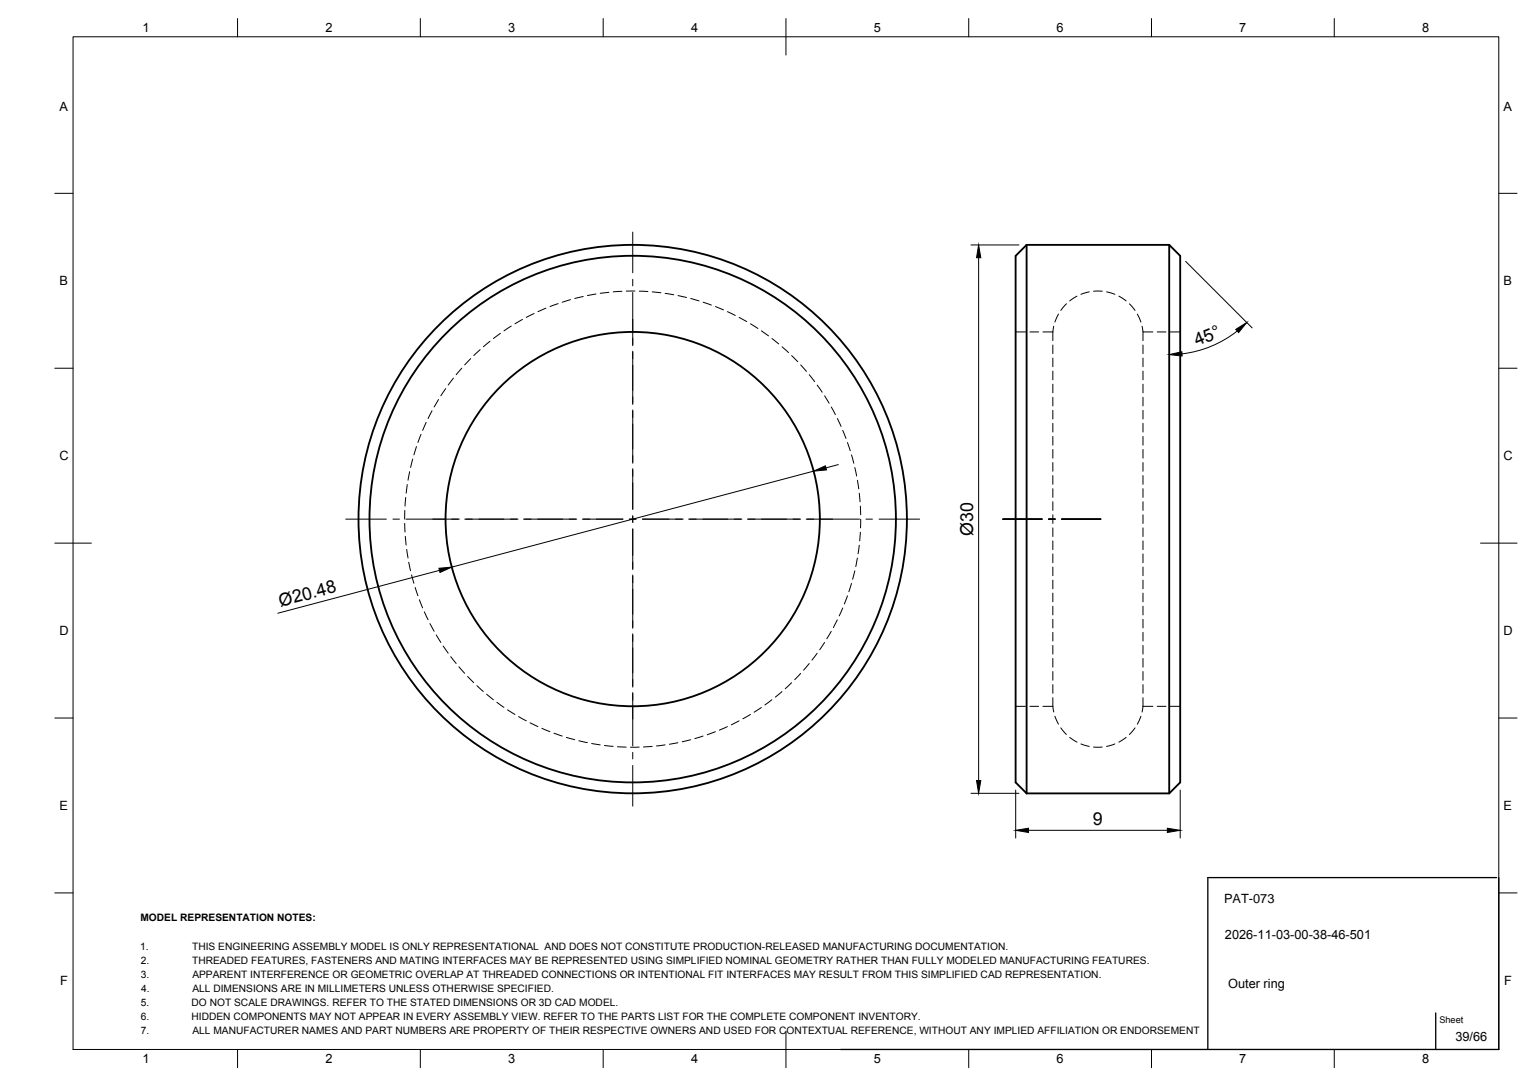
ISO-10303-21;
HEADER;
/* Generated by software containing ST-Developer
 * from STEP Tools, Inc. (www.steptools.com) 
 */

FILE_DESCRIPTION(
/* description */ ('Manual piston pump'),
/* implementation_level */ '2;1');

FILE_NAME(
/* name */ 'Outer ring.step',
/* time_stamp */ '2026-11-02T16:54:23-08:00',
/* author */ (''),
/* organization */ (''),
/* preprocessor_version */ 'ST-DEVELOPER v20.2',
/* originating_system */ 'Autodesk Translation Framework v15.17.0.0',
/* authorisation */ '');

FILE_SCHEMA (('AUTOMOTIVE_DESIGN { 1 0 10303 214 3 1 1 }'));
ENDSEC;

DATA;
#10=MECHANICAL_DESIGN_GEOMETRIC_PRESENTATION_REPRESENTATION('',(#712),#19043);
#539=CONICAL_SURFACE('',#10737,1.47,0.785398163397449);
#540=CONICAL_SURFACE('',#10741,1.47,0.785398163397449);
#560=TOROIDAL_SURFACE('',#10726,1.,0.247676);
#586=SHAPE_REPRESENTATION_RELATIONSHIP('SRR','None',#19333,#649);
#649=ADVANCED_BREP_SHAPE_REPRESENTATION('',(#782),#19000);
#712=STYLED_ITEM('',(#19664),#782);
#782=MANIFOLD_SOLID_BREP('Body1',#9498);
#948=FACE_BOUND('',#2237,.T.);
#949=FACE_BOUND('',#2242,.T.);
#1186=CYLINDRICAL_SURFACE('',#10732,1.023815);
#1187=CYLINDRICAL_SURFACE('',#10739,1.5);
#1188=CYLINDRICAL_SURFACE('',#10744,1.023815);
#1538=FACE_OUTER_BOUND('',#2234,.T.);
#1539=FACE_OUTER_BOUND('',#2235,.T.);
#1540=FACE_OUTER_BOUND('',#2236,.T.);
#1541=FACE_OUTER_BOUND('',#2238,.T.);
#1542=FACE_OUTER_BOUND('',#2239,.T.);
#1543=FACE_OUTER_BOUND('',#2240,.T.);
#1544=FACE_OUTER_BOUND('',#2241,.T.);
#1545=FACE_OUTER_BOUND('',#2243,.T.);
#2234=EDGE_LOOP('',(#7281,#7282,#7283,#7284,#7285,#7286));
#2235=EDGE_LOOP('',(#7287,#7288,#7289,#7290,#7291));
#2236=EDGE_LOOP('',(#7292));
#2237=EDGE_LOOP('',(#7293));
#2238=EDGE_LOOP('',(#7294,#7295,#7296,#7297));
#2239=EDGE_LOOP('',(#7298,#7299,#7300,#7301));
#2240=EDGE_LOOP('',(#7302,#7303,#7304,#7305));
#2241=EDGE_LOOP('',(#7306));
#2242=EDGE_LOOP('',(#7307));
#2243=EDGE_LOOP('',(#7308,#7309,#7310,#7311,#7312));
#2872=CIRCLE('',#10727,1.023815);
#2873=CIRCLE('',#10728,1.023815);
#2874=CIRCLE('',#10729,0.247676);
#2875=CIRCLE('',#10730,1.023815);
#2876=CIRCLE('',#10731,1.023815);
#2877=CIRCLE('',#10733,1.023815);
#2878=CIRCLE('',#10735,1.44);
#2879=CIRCLE('',#10736,1.023815);
#2880=CIRCLE('',#10738,1.5);
#2881=CIRCLE('',#10740,1.5);
#2882=CIRCLE('',#10742,1.44);
#3427=LINE('',#15800,#4031);
#3428=LINE('',#15809,#4032);
#3429=LINE('',#15813,#4033);
#3430=LINE('',#15817,#4034);
#3431=LINE('',#15820,#4035);
#4031=VECTOR('',#12757,1.023815);
#4032=VECTOR('',#12768,1.47);
#4033=VECTOR('',#12773,1.5);
#4034=VECTOR('',#12778,1.47);
#4035=VECTOR('',#12783,1.023815);
#4686=VERTEX_POINT('',#15788);
#4687=VERTEX_POINT('',#15789);
#4688=VERTEX_POINT('',#15792);
#4689=VERTEX_POINT('',#15794);
#4690=VERTEX_POINT('',#15798);
#4691=VERTEX_POINT('',#15802);
#4692=VERTEX_POINT('',#15804);
#4693=VERTEX_POINT('',#15807);
#4694=VERTEX_POINT('',#15811);
#4695=VERTEX_POINT('',#15815);
#5627=EDGE_CURVE('',#4686,#4687,#2872,.T.);
#5628=EDGE_CURVE('',#4687,#4686,#2873,.T.);
#5629=EDGE_CURVE('',#4687,#4688,#2874,.T.);
#5630=EDGE_CURVE('',#4689,#4688,#2875,.T.);
#5631=EDGE_CURVE('',#4688,#4689,#2876,.T.);
#5632=EDGE_CURVE('',#4690,#4690,#2877,.T.);
#5633=EDGE_CURVE('',#4690,#4689,#3427,.T.);
#5634=EDGE_CURVE('',#4691,#4691,#2878,.T.);
#5635=EDGE_CURVE('',#4692,#4692,#2879,.T.);
#5636=EDGE_CURVE('',#4693,#4693,#2880,.T.);
#5637=EDGE_CURVE('',#4693,#4691,#3428,.T.);
#5638=EDGE_CURVE('',#4694,#4694,#2881,.T.);
#5639=EDGE_CURVE('',#4694,#4693,#3429,.T.);
#5640=EDGE_CURVE('',#4695,#4695,#2882,.T.);
#5641=EDGE_CURVE('',#4695,#4694,#3430,.T.);
#5642=EDGE_CURVE('',#4686,#4692,#3431,.T.);
#7281=ORIENTED_EDGE('',*,*,#5627,.F.);
#7282=ORIENTED_EDGE('',*,*,#5628,.F.);
#7283=ORIENTED_EDGE('',*,*,#5629,.T.);
#7284=ORIENTED_EDGE('',*,*,#5630,.F.);
#7285=ORIENTED_EDGE('',*,*,#5631,.F.);
#7286=ORIENTED_EDGE('',*,*,#5629,.F.);
#7287=ORIENTED_EDGE('',*,*,#5632,.T.);
#7288=ORIENTED_EDGE('',*,*,#5633,.T.);
#7289=ORIENTED_EDGE('',*,*,#5630,.T.);
#7290=ORIENTED_EDGE('',*,*,#5631,.T.);
#7291=ORIENTED_EDGE('',*,*,#5633,.F.);
#7292=ORIENTED_EDGE('',*,*,#5634,.F.);
#7293=ORIENTED_EDGE('',*,*,#5635,.T.);
#7294=ORIENTED_EDGE('',*,*,#5636,.F.);
#7295=ORIENTED_EDGE('',*,*,#5637,.T.);
#7296=ORIENTED_EDGE('',*,*,#5634,.T.);
#7297=ORIENTED_EDGE('',*,*,#5637,.F.);
#7298=ORIENTED_EDGE('',*,*,#5638,.F.);
#7299=ORIENTED_EDGE('',*,*,#5639,.T.);
#7300=ORIENTED_EDGE('',*,*,#5636,.T.);
#7301=ORIENTED_EDGE('',*,*,#5639,.F.);
#7302=ORIENTED_EDGE('',*,*,#5640,.F.);
#7303=ORIENTED_EDGE('',*,*,#5641,.T.);
#7304=ORIENTED_EDGE('',*,*,#5638,.T.);
#7305=ORIENTED_EDGE('',*,*,#5641,.F.);
#7306=ORIENTED_EDGE('',*,*,#5640,.T.);
#7307=ORIENTED_EDGE('',*,*,#5632,.F.);
#7308=ORIENTED_EDGE('',*,*,#5627,.T.);
#7309=ORIENTED_EDGE('',*,*,#5628,.T.);
#7310=ORIENTED_EDGE('',*,*,#5642,.T.);
#7311=ORIENTED_EDGE('',*,*,#5635,.F.);
#7312=ORIENTED_EDGE('',*,*,#5642,.F.);
#8710=PLANE('',#10734);
#8711=PLANE('',#10743);
#9143=ADVANCED_FACE('',(#1538),#560,.F.);
#9144=ADVANCED_FACE('',(#1539),#1186,.F.);
#9145=ADVANCED_FACE('',(#1540,#948),#8710,.T.);
#9146=ADVANCED_FACE('',(#1541),#539,.T.);
#9147=ADVANCED_FACE('',(#1542),#1187,.T.);
#9148=ADVANCED_FACE('',(#1543),#540,.T.);
#9149=ADVANCED_FACE('',(#1544,#949),#8711,.T.);
#9150=ADVANCED_FACE('',(#1545),#1188,.F.);
#9498=CLOSED_SHELL('',(#9143,#9144,#9145,#9146,#9147,#9148,#9149,#9150));
#10725=AXIS2_PLACEMENT_3D('',#15786,#12739,#12740);
#10726=AXIS2_PLACEMENT_3D('',#15787,#12741,#12742);
#10727=AXIS2_PLACEMENT_3D('',#15790,#12743,#12744);
#10728=AXIS2_PLACEMENT_3D('',#15791,#12745,#12746);
#10729=AXIS2_PLACEMENT_3D('',#15793,#12747,#12748);
#10730=AXIS2_PLACEMENT_3D('',#15795,#12749,#12750);
#10731=AXIS2_PLACEMENT_3D('',#15796,#12751,#12752);
#10732=AXIS2_PLACEMENT_3D('',#15797,#12753,#12754);
#10733=AXIS2_PLACEMENT_3D('',#15799,#12755,#12756);
#10734=AXIS2_PLACEMENT_3D('',#15801,#12758,#12759);
#10735=AXIS2_PLACEMENT_3D('',#15803,#12760,#12761);
#10736=AXIS2_PLACEMENT_3D('',#15805,#12762,#12763);
#10737=AXIS2_PLACEMENT_3D('',#15806,#12764,#12765);
#10738=AXIS2_PLACEMENT_3D('',#15808,#12766,#12767);
#10739=AXIS2_PLACEMENT_3D('',#15810,#12769,#12770);
#10740=AXIS2_PLACEMENT_3D('',#15812,#12771,#12772);
#10741=AXIS2_PLACEMENT_3D('',#15814,#12774,#12775);
#10742=AXIS2_PLACEMENT_3D('',#15816,#12776,#12777);
#10743=AXIS2_PLACEMENT_3D('',#15818,#12779,#12780);
#10744=AXIS2_PLACEMENT_3D('',#15819,#12781,#12782);
#12739=DIRECTION('axis',(0.,0.,1.));
#12740=DIRECTION('refdir',(1.,0.,0.));
#12741=DIRECTION('center_axis',(0.,-1.,0.));
#12742=DIRECTION('ref_axis',(0.,0.,-1.));
#12743=DIRECTION('center_axis',(0.,-1.,0.));
#12744=DIRECTION('ref_axis',(1.,0.,0.));
#12745=DIRECTION('center_axis',(0.,-1.,0.));
#12746=DIRECTION('ref_axis',(1.,0.,0.));
#12747=DIRECTION('center_axis',(1.,0.,1.22464679914735E-16));
#12748=DIRECTION('ref_axis',(-1.22464679914735E-16,0.,1.));
#12749=DIRECTION('center_axis',(0.,1.,0.));
#12750=DIRECTION('ref_axis',(1.,0.,0.));
#12751=DIRECTION('center_axis',(0.,1.,0.));
#12752=DIRECTION('ref_axis',(1.,0.,0.));
#12753=DIRECTION('center_axis',(0.,-1.,0.));
#12754=DIRECTION('ref_axis',(1.,0.,0.));
#12755=DIRECTION('center_axis',(0.,-1.,0.));
#12756=DIRECTION('ref_axis',(1.,0.,0.));
#12757=DIRECTION('',(0.,1.,0.));
#12758=DIRECTION('center_axis',(0.,1.,0.));
#12759=DIRECTION('ref_axis',(0.,0.,1.));
#12760=DIRECTION('center_axis',(0.,-1.,0.));
#12761=DIRECTION('ref_axis',(1.,0.,0.));
#12762=DIRECTION('center_axis',(0.,-1.,0.));
#12763=DIRECTION('ref_axis',(1.,0.,0.));
#12764=DIRECTION('center_axis',(0.,-1.,0.));
#12765=DIRECTION('ref_axis',(1.,0.,0.));
#12766=DIRECTION('center_axis',(0.,-1.,0.));
#12767=DIRECTION('ref_axis',(1.,0.,0.));
#12768=DIRECTION('',(0.707106781186548,0.707106781186547,8.65956056235494E-17));
#12769=DIRECTION('center_axis',(0.,-1.,0.));
#12770=DIRECTION('ref_axis',(1.,0.,0.));
#12771=DIRECTION('center_axis',(0.,-1.,0.));
#12772=DIRECTION('ref_axis',(1.,0.,0.));
#12773=DIRECTION('',(0.,1.,0.));
#12774=DIRECTION('center_axis',(0.,1.,0.));
#12775=DIRECTION('ref_axis',(1.,0.,0.));
#12776=DIRECTION('center_axis',(0.,-1.,0.));
#12777=DIRECTION('ref_axis',(1.,0.,0.));
#12778=DIRECTION('',(-0.707106781186548,0.707106781186547,-8.65956056235494E-17));
#12779=DIRECTION('center_axis',(0.,-1.,0.));
#12780=DIRECTION('ref_axis',(0.,0.,-1.));
#12781=DIRECTION('center_axis',(0.,-1.,0.));
#12782=DIRECTION('ref_axis',(1.,0.,0.));
#12783=DIRECTION('',(0.,1.,0.));
#15786=CARTESIAN_POINT('',(0.,0.,0.));
#15787=CARTESIAN_POINT('Origin',(0.,0.,0.));
#15788=CARTESIAN_POINT('',(-1.023815,0.246528389340863,-1.25381176266905E-16));
#15789=CARTESIAN_POINT('',(-1.25381176266905E-16,0.246528389340863,1.023815));
#15790=CARTESIAN_POINT('Origin',(0.,0.246528389340863,0.));
#15791=CARTESIAN_POINT('Origin',(0.,0.246528389340863,0.));
#15792=CARTESIAN_POINT('',(-1.25381176266905E-16,-0.246528389340863,1.023815));
#15793=CARTESIAN_POINT('Origin',(-1.22464679914735E-16,0.,1.));
#15794=CARTESIAN_POINT('',(-1.023815,-0.246528389340863,1.25381176266905E-16));
#15795=CARTESIAN_POINT('Origin',(0.,-0.246528389340863,0.));
#15796=CARTESIAN_POINT('Origin',(0.,-0.246528389340863,0.));
#15797=CARTESIAN_POINT('Origin',(0.,0.,0.));
#15798=CARTESIAN_POINT('',(-1.023815,-0.45,-1.25381176266905E-16));
#15799=CARTESIAN_POINT('Origin',(0.,-0.45,0.));
#15800=CARTESIAN_POINT('',(-1.023815,0.,-1.25381176266905E-16));
#15801=CARTESIAN_POINT('Origin',(1.44,0.45,0.));
#15802=CARTESIAN_POINT('',(-1.44,0.45,-1.76349139077219E-16));
#15803=CARTESIAN_POINT('Origin',(0.,0.45,0.));
#15804=CARTESIAN_POINT('',(-1.023815,0.45,-1.25381176266905E-16));
#15805=CARTESIAN_POINT('Origin',(0.,0.45,0.));
#15806=CARTESIAN_POINT('Origin',(0.,0.42,0.));
#15807=CARTESIAN_POINT('',(-1.5,0.39,-1.83697019872103E-16));
#15808=CARTESIAN_POINT('Origin',(0.,0.39,0.));
#15809=CARTESIAN_POINT('',(-1.47,0.42,-1.80023079474661E-16));
#15810=CARTESIAN_POINT('Origin',(0.,0.,0.));
#15811=CARTESIAN_POINT('',(-1.5,-0.39,-1.83697019872103E-16));
#15812=CARTESIAN_POINT('Origin',(0.,-0.39,0.));
#15813=CARTESIAN_POINT('',(-1.5,0.,-1.83697019872103E-16));
#15814=CARTESIAN_POINT('Origin',(0.,-0.42,0.));
#15815=CARTESIAN_POINT('',(-1.44,-0.45,-1.76349139077219E-16));
#15816=CARTESIAN_POINT('Origin',(0.,-0.45,0.));
#15817=CARTESIAN_POINT('',(-1.47,-0.42,-1.80023079474661E-16));
#15818=CARTESIAN_POINT('Origin',(1.023815,-0.45,0.));
#15819=CARTESIAN_POINT('Origin',(0.,0.,0.));
#15820=CARTESIAN_POINT('',(-1.023815,0.,-1.25381176266905E-16));
#18929=UNCERTAINTY_MEASURE_WITH_UNIT(LENGTH_MEASURE(0.001),#19044,
'DISTANCE_ACCURACY_VALUE',
'Maximum model space distance between geometric entities at asserted c
onnectivities');
#18972=UNCERTAINTY_MEASURE_WITH_UNIT(LENGTH_MEASURE(0.001),#19044,
'DISTANCE_ACCURACY_VALUE',
'Maximum model space distance between geometric entities at asserted c
onnectivities');
#19000=(
GEOMETRIC_REPRESENTATION_CONTEXT(3)
GLOBAL_UNCERTAINTY_ASSIGNED_CONTEXT((#18929))
GLOBAL_UNIT_ASSIGNED_CONTEXT((#19044,#19046,#19047))
REPRESENTATION_CONTEXT('','3D')
);
#19043=(
GEOMETRIC_REPRESENTATION_CONTEXT(3)
GLOBAL_UNCERTAINTY_ASSIGNED_CONTEXT((#18972))
GLOBAL_UNIT_ASSIGNED_CONTEXT((#19044,#19046,#19047))
REPRESENTATION_CONTEXT('','3D')
);
#19044=(
LENGTH_UNIT()
NAMED_UNIT(*)
SI_UNIT(.CENTI.,.METRE.)
);
#19046=(
NAMED_UNIT(*)
PLANE_ANGLE_UNIT()
SI_UNIT($,.RADIAN.)
);
#19047=(
NAMED_UNIT(*)
SI_UNIT($,.STERADIAN.)
SOLID_ANGLE_UNIT()
);
#19075=SHAPE_DEFINITION_REPRESENTATION(#19145,#19333);
#19145=PRODUCT_DEFINITION_SHAPE('',$,#19404);
#19333=SHAPE_REPRESENTATION('',(#10725),#19000);
#19376=PRODUCT_DEFINITION_CONTEXT('part definition',#19588,'design');
#19404=PRODUCT_DEFINITION('2026-11-03-00-38-46-501','Outer ring',#19474,
#19376);
#19474=PRODUCT_DEFINITION_FORMATION('',$,#19617);
#19588=APPLICATION_CONTEXT(
'Core Data for Automotive Mechanical Design Process');
#19589=PRODUCT_CONTEXT('part definition',#19588,'mechanical');
#19617=PRODUCT('2026-11-03-00-38-46-501','Outer ring','Outer ring',(#19589));
#19664=PRESENTATION_STYLE_ASSIGNMENT((#19670));
#19670=SURFACE_STYLE_USAGE(.BOTH.,#19676);
#19676=SURFACE_SIDE_STYLE('',(#19682));
#19682=SURFACE_STYLE_FILL_AREA(#19688);
#19688=FILL_AREA_STYLE('CAD Library Painted - Steel gray',(#19694));
#19694=FILL_AREA_STYLE_COLOUR('CAD Library Painted - Steel gray',#19700);
#19700=COLOUR_RGB('CAD Library Painted - Steel gray',0.592156862745098,
0.631372549019608,0.67843137254902);
ENDSEC;
END-ISO-10303-21;
